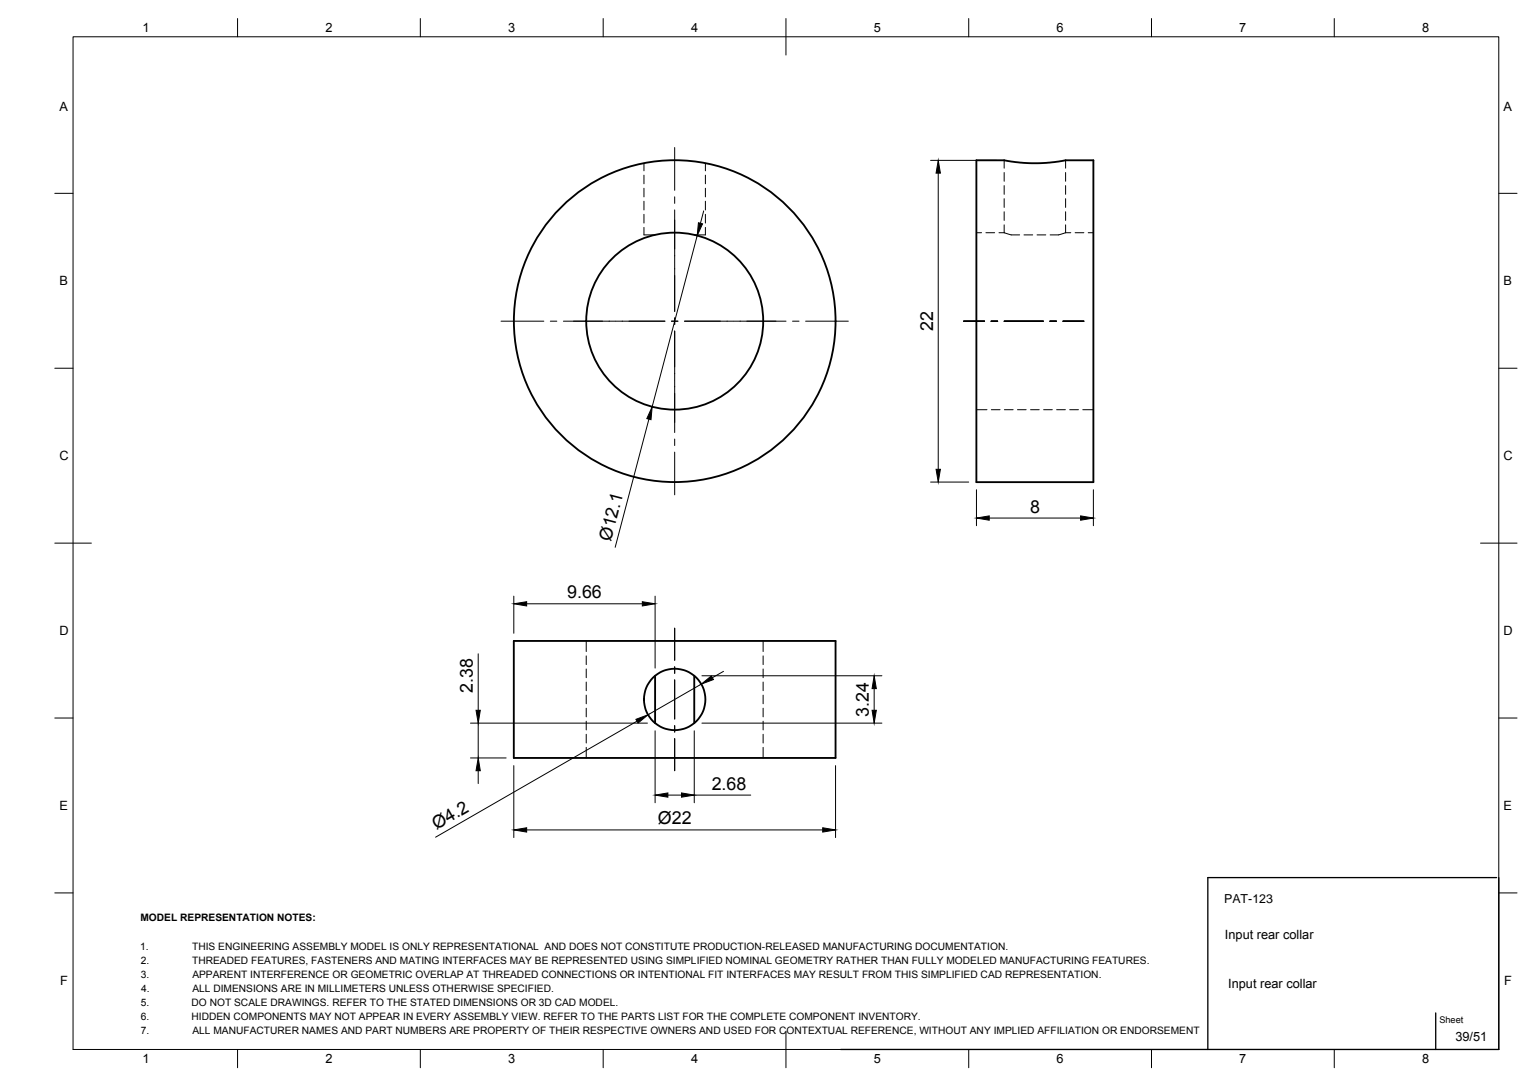
ISO-10303-21;
HEADER;
/* Generated by software containing ST-Developer
 * from STEP Tools, Inc. (www.steptools.com) 
 */

FILE_DESCRIPTION(
/* description */ ('Worm-less right-angle friction wheel drive'),
/* implementation_level */ '2;1');

FILE_NAME(
/* name */ 'Input rear collar.step',
/* time_stamp */ '2026-10-28T03:22:36-07:00',
/* author */ (''),
/* organization */ (''),
/* preprocessor_version */ 'ST-DEVELOPER v20.2',
/* originating_system */ 'Autodesk Translation Framework v15.17.0.0',
/* authorisation */ '');

FILE_SCHEMA (('AUTOMOTIVE_DESIGN { 1 0 10303 214 3 1 1 }'));
ENDSEC;

DATA;
#10=MECHANICAL_DESIGN_GEOMETRIC_PRESENTATION_REPRESENTATION('',(#652),#17046);
#497=B_SPLINE_CURVE_WITH_KNOTS('',3,(#16212,#16213,#16214,#16215,#16216,
#16217,#16218,#16219,#16220,#16221),.UNSPECIFIED.,.F.,.F.,(4,2,2,2,4),(0.818088904349172,
0.878131747417165,0.957937926194036,1.03774410497091,1.0977869480389),
 .UNSPECIFIED.);
#498=B_SPLINE_CURVE_WITH_KNOTS('',3,(#16227,#16228,#16229,#16230,#16231,
#16232,#16233,#16234,#16235,#16236,#16237,#16238,#16239,#16240,#16241,#16242,
#16243,#16244),.UNSPECIFIED.,.F.,.F.,(4,2,2,2,2,2,2,2,4),(0.,0.0793157643915219,
0.158631528783044,0.23794361593365,0.317255703084256,0.396567790234861,
0.475879877385467,0.555195641776989,0.634511406168511),.UNSPECIFIED.);
#499=B_SPLINE_CURVE_WITH_KNOTS('',3,(#16245,#16246,#16247,#16248,#16249,
#16250,#16251,#16252,#16253,#16254,#16255,#16256,#16257,#16258,#16259,#16260,
#16261,#16262),.UNSPECIFIED.,.F.,.F.,(4,2,2,2,2,2,2,2,4),(0.634511406168511,
0.713827170560033,0.793142934951555,0.872455022102161,0.951767109252766,
1.03107919640337,1.11039128355398,1.1897070479455,1.26902281233702),
 .UNSPECIFIED.);
#500=B_SPLINE_CURVE_WITH_KNOTS('',3,(#16265,#16266,#16267,#16268,#16269,
#16270,#16271,#16272,#16273,#16274),.UNSPECIFIED.,.F.,.F.,(4,2,2,2,4),(0.179463620219816,
0.239506463287808,0.319312642064679,0.399118820841549,0.459161663909541),
 .UNSPECIFIED.);
#551=SHAPE_REPRESENTATION_RELATIONSHIP('SRR','None',#17296,#598);
#598=ADVANCED_BREP_SHAPE_REPRESENTATION('',(#703),#17032);
#652=STYLED_ITEM('',(#17584),#703);
#703=MANIFOLD_SOLID_BREP('Body1',#8210);
#925=FACE_BOUND('',#2249,.T.);
#926=FACE_BOUND('',#2251,.T.);
#927=FACE_BOUND('',#2253,.T.);
#928=FACE_BOUND('',#2255,.T.);
#1137=PLANE('',#9491);
#1138=PLANE('',#9496);
#1139=PLANE('',#9503);
#1140=PLANE('',#9504);
#1569=FACE_OUTER_BOUND('',#2245,.T.);
#1570=FACE_OUTER_BOUND('',#2246,.T.);
#1571=FACE_OUTER_BOUND('',#2247,.T.);
#1572=FACE_OUTER_BOUND('',#2248,.T.);
#1573=FACE_OUTER_BOUND('',#2250,.T.);
#1574=FACE_OUTER_BOUND('',#2252,.T.);
#1575=FACE_OUTER_BOUND('',#2254,.T.);
#2245=EDGE_LOOP('',(#7098,#7099));
#2246=EDGE_LOOP('',(#7100,#7101,#7102,#7103,#7104,#7105,#7106,#7107,#7108));
#2247=EDGE_LOOP('',(#7109,#7110,#7111));
#2248=EDGE_LOOP('',(#7112,#7113,#7114,#7115));
#2249=EDGE_LOOP('',(#7116,#7117,#7118,#7119));
#2250=EDGE_LOOP('',(#7120,#7121,#7122,#7123));
#2251=EDGE_LOOP('',(#7124,#7125));
#2252=EDGE_LOOP('',(#7126));
#2253=EDGE_LOOP('',(#7127));
#2254=EDGE_LOOP('',(#7128));
#2255=EDGE_LOOP('',(#7129));
#2785=LINE('',#16208,#3325);
#2786=LINE('',#16225,#3326);
#2787=LINE('',#16276,#3327);
#2788=LINE('',#16281,#3328);
#2789=LINE('',#16287,#3329);
#3325=VECTOR('',#11681,1.);
#3326=VECTOR('',#11688,0.21);
#3327=VECTOR('',#11693,1.);
#3328=VECTOR('',#11698,0.605);
#3329=VECTOR('',#11705,1.1);
#3803=CIRCLE('',#9492,0.21);
#3804=CIRCLE('',#9494,0.21);
#3805=CIRCLE('',#9495,0.21);
#3806=CIRCLE('',#9498,0.605);
#3807=CIRCLE('',#9499,0.605);
#3808=CIRCLE('',#9501,1.1);
#3809=CIRCLE('',#9502,1.1);
#4394=VERTEX_POINT('',#16206);
#4395=VERTEX_POINT('',#16207);
#4396=VERTEX_POINT('',#16211);
#4397=VERTEX_POINT('',#16222);
#4398=VERTEX_POINT('',#16224);
#4399=VERTEX_POINT('',#16226);
#4400=VERTEX_POINT('',#16263);
#4401=VERTEX_POINT('',#16278);
#4402=VERTEX_POINT('',#16280);
#4403=VERTEX_POINT('',#16284);
#4404=VERTEX_POINT('',#16286);
#5318=EDGE_CURVE('',#4394,#4395,#2785,.T.);
#5319=EDGE_CURVE('',#4394,#4395,#3803,.T.);
#5320=EDGE_CURVE('',#4396,#4394,#497,.T.);
#5321=EDGE_CURVE('',#4397,#4396,#3804,.T.);
#5322=EDGE_CURVE('',#4397,#4398,#2786,.T.);
#5323=EDGE_CURVE('',#4399,#4398,#498,.T.);
#5324=EDGE_CURVE('',#4398,#4399,#499,.T.);
#5325=EDGE_CURVE('',#4400,#4397,#3805,.T.);
#5326=EDGE_CURVE('',#4395,#4400,#500,.T.);
#5327=EDGE_CURVE('',#4400,#4396,#2787,.T.);
#5328=EDGE_CURVE('',#4401,#4401,#3806,.T.);
#5329=EDGE_CURVE('',#4401,#4402,#2788,.T.);
#5330=EDGE_CURVE('',#4402,#4402,#3807,.T.);
#5331=EDGE_CURVE('',#4403,#4403,#3808,.T.);
#5332=EDGE_CURVE('',#4403,#4404,#2789,.T.);
#5333=EDGE_CURVE('',#4404,#4404,#3809,.T.);
#7098=ORIENTED_EDGE('',*,*,#5318,.F.);
#7099=ORIENTED_EDGE('',*,*,#5319,.T.);
#7100=ORIENTED_EDGE('',*,*,#5320,.F.);
#7101=ORIENTED_EDGE('',*,*,#5321,.F.);
#7102=ORIENTED_EDGE('',*,*,#5322,.T.);
#7103=ORIENTED_EDGE('',*,*,#5323,.F.);
#7104=ORIENTED_EDGE('',*,*,#5324,.F.);
#7105=ORIENTED_EDGE('',*,*,#5322,.F.);
#7106=ORIENTED_EDGE('',*,*,#5325,.F.);
#7107=ORIENTED_EDGE('',*,*,#5326,.F.);
#7108=ORIENTED_EDGE('',*,*,#5319,.F.);
#7109=ORIENTED_EDGE('',*,*,#5327,.F.);
#7110=ORIENTED_EDGE('',*,*,#5325,.T.);
#7111=ORIENTED_EDGE('',*,*,#5321,.T.);
#7112=ORIENTED_EDGE('',*,*,#5328,.F.);
#7113=ORIENTED_EDGE('',*,*,#5329,.T.);
#7114=ORIENTED_EDGE('',*,*,#5330,.T.);
#7115=ORIENTED_EDGE('',*,*,#5329,.F.);
#7116=ORIENTED_EDGE('',*,*,#5326,.T.);
#7117=ORIENTED_EDGE('',*,*,#5327,.T.);
#7118=ORIENTED_EDGE('',*,*,#5320,.T.);
#7119=ORIENTED_EDGE('',*,*,#5318,.T.);
#7120=ORIENTED_EDGE('',*,*,#5331,.F.);
#7121=ORIENTED_EDGE('',*,*,#5332,.T.);
#7122=ORIENTED_EDGE('',*,*,#5333,.T.);
#7123=ORIENTED_EDGE('',*,*,#5332,.F.);
#7124=ORIENTED_EDGE('',*,*,#5323,.T.);
#7125=ORIENTED_EDGE('',*,*,#5324,.T.);
#7126=ORIENTED_EDGE('',*,*,#5331,.T.);
#7127=ORIENTED_EDGE('',*,*,#5328,.T.);
#7128=ORIENTED_EDGE('',*,*,#5333,.F.);
#7129=ORIENTED_EDGE('',*,*,#5330,.F.);
#7671=CYLINDRICAL_SURFACE('',#9493,0.21);
#7672=CYLINDRICAL_SURFACE('',#9497,0.605);
#7673=CYLINDRICAL_SURFACE('',#9500,1.1);
#8061=ADVANCED_FACE('',(#1569),#1137,.T.);
#8062=ADVANCED_FACE('',(#1570),#7671,.F.);
#8063=ADVANCED_FACE('',(#1571),#1138,.T.);
#8064=ADVANCED_FACE('',(#1572,#925),#7672,.F.);
#8065=ADVANCED_FACE('',(#1573,#926),#7673,.T.);
#8066=ADVANCED_FACE('',(#1574,#927),#1139,.T.);
#8067=ADVANCED_FACE('',(#1575,#928),#1140,.F.);
#8210=CLOSED_SHELL('',(#8061,#8062,#8063,#8064,#8065,#8066,#8067));
#9490=AXIS2_PLACEMENT_3D('',#16204,#11677,#11678);
#9491=AXIS2_PLACEMENT_3D('',#16205,#11679,#11680);
#9492=AXIS2_PLACEMENT_3D('',#16209,#11682,#11683);
#9493=AXIS2_PLACEMENT_3D('',#16210,#11684,#11685);
#9494=AXIS2_PLACEMENT_3D('',#16223,#11686,#11687);
#9495=AXIS2_PLACEMENT_3D('',#16264,#11689,#11690);
#9496=AXIS2_PLACEMENT_3D('',#16275,#11691,#11692);
#9497=AXIS2_PLACEMENT_3D('',#16277,#11694,#11695);
#9498=AXIS2_PLACEMENT_3D('',#16279,#11696,#11697);
#9499=AXIS2_PLACEMENT_3D('',#16282,#11699,#11700);
#9500=AXIS2_PLACEMENT_3D('',#16283,#11701,#11702);
#9501=AXIS2_PLACEMENT_3D('',#16285,#11703,#11704);
#9502=AXIS2_PLACEMENT_3D('',#16288,#11706,#11707);
#9503=AXIS2_PLACEMENT_3D('',#16289,#11708,#11709);
#9504=AXIS2_PLACEMENT_3D('',#16290,#11710,#11711);
#11677=DIRECTION('axis',(0.,0.,1.));
#11678=DIRECTION('refdir',(1.,0.,0.));
#11679=DIRECTION('center_axis',(0.,0.,1.));
#11680=DIRECTION('ref_axis',(1.,0.,0.));
#11681=DIRECTION('',(0.,1.,0.));
#11682=DIRECTION('center_axis',(0.,0.,1.));
#11683=DIRECTION('ref_axis',(1.,0.,0.));
#11684=DIRECTION('center_axis',(0.,0.,1.));
#11685=DIRECTION('ref_axis',(1.,0.,0.));
#11686=DIRECTION('center_axis',(0.,0.,1.));
#11687=DIRECTION('ref_axis',(1.,0.,0.));
#11688=DIRECTION('',(0.,0.,1.));
#11689=DIRECTION('center_axis',(0.,0.,1.));
#11690=DIRECTION('ref_axis',(1.,0.,0.));
#11691=DIRECTION('center_axis',(0.,0.,1.));
#11692=DIRECTION('ref_axis',(1.,0.,0.));
#11693=DIRECTION('',(0.,-1.,0.));
#11694=DIRECTION('center_axis',(0.,1.,0.));
#11695=DIRECTION('ref_axis',(1.,0.,0.));
#11696=DIRECTION('center_axis',(0.,-1.,0.));
#11697=DIRECTION('ref_axis',(1.,0.,0.));
#11698=DIRECTION('',(0.,-1.,0.));
#11699=DIRECTION('center_axis',(0.,-1.,0.));
#11700=DIRECTION('ref_axis',(1.,0.,0.));
#11701=DIRECTION('center_axis',(0.,1.,0.));
#11702=DIRECTION('ref_axis',(1.,0.,0.));
#11703=DIRECTION('center_axis',(0.,1.,0.));
#11704=DIRECTION('ref_axis',(1.,0.,0.));
#11705=DIRECTION('',(0.,-1.,0.));
#11706=DIRECTION('center_axis',(0.,1.,0.));
#11707=DIRECTION('ref_axis',(1.,0.,0.));
#11708=DIRECTION('center_axis',(0.,1.,0.));
#11709=DIRECTION('ref_axis',(1.,0.,0.));
#11710=DIRECTION('center_axis',(0.,1.,0.));
#11711=DIRECTION('ref_axis',(1.,0.,0.));
#16204=CARTESIAN_POINT('',(0.,0.,0.));
#16205=CARTESIAN_POINT('Origin',(0.,-7.9,7.59));
#16206=CARTESIAN_POINT('',(0.133884278389956,-8.06178689687364,7.59));
#16207=CARTESIAN_POINT('',(0.133884278389956,-7.73821310312636,7.59));
#16208=CARTESIAN_POINT('',(0.133884278389956,-8.3,7.59));
#16209=CARTESIAN_POINT('Origin',(0.,-7.9,7.59));
#16210=CARTESIAN_POINT('Origin',(0.,-7.9,7.59));
#16211=CARTESIAN_POINT('',(-0.133884278389956,-8.06178689687364,7.59));
#16212=CARTESIAN_POINT('Ctrl Pts',(-0.133884278389956,-8.06178689687364,
7.59));
#16213=CARTESIAN_POINT('Ctrl Pts',(-0.118254395260802,-8.07472116821763,
7.59354677224418));
#16214=CARTESIAN_POINT('Ctrl Pts',(-0.100109787682299,-8.08579931658744,
7.59698224789957));
#16215=CARTESIAN_POINT('Ctrl Pts',(-0.054829872132519,-8.10463856105443,
7.6030741628997));
#16216=CARTESIAN_POINT('Ctrl Pts',(-0.0266020595922904,-8.11,7.605));
#16217=CARTESIAN_POINT('Ctrl Pts',(0.0266020595922903,-8.11,7.605));
#16218=CARTESIAN_POINT('Ctrl Pts',(0.0548298721325189,-8.10463856105443,
7.6030741628997));
#16219=CARTESIAN_POINT('Ctrl Pts',(0.100109787682299,-8.08579931658744,
7.59698224789957));
#16220=CARTESIAN_POINT('Ctrl Pts',(0.118254395260802,-8.07472116821763,
7.59354677224418));
#16221=CARTESIAN_POINT('Ctrl Pts',(0.133884278389957,-8.06178689687364,
7.59));
#16222=CARTESIAN_POINT('',(-0.21,-7.9,7.59));
#16223=CARTESIAN_POINT('Origin',(0.,-7.9,7.59));
#16224=CARTESIAN_POINT('',(-0.21,-7.9,8.07976849370594));
#16225=CARTESIAN_POINT('',(-0.21,-7.9,7.59));
#16226=CARTESIAN_POINT('',(0.21,-7.9,8.07976849370594));
#16227=CARTESIAN_POINT('Ctrl Pts',(0.21,-7.9,8.07976849370594));
#16228=CARTESIAN_POINT('Ctrl Pts',(0.21,-7.92643858813051,8.07976849370594));
#16229=CARTESIAN_POINT('Ctrl Pts',(0.204702922670977,-7.95459378125493,
8.08084015664674));
#16230=CARTESIAN_POINT('Ctrl Pts',(0.183251796806355,-8.00631344554134,
8.08468313707126));
#16231=CARTESIAN_POINT('Ctrl Pts',(0.167101177357214,-8.02988367074114,
8.08739593054622));
#16232=CARTESIAN_POINT('Ctrl Pts',(0.129884533480965,-8.06710031461738,
8.09246633289124));
#16233=CARTESIAN_POINT('Ctrl Pts',(0.106313940757289,-8.08325161016341,
8.09515738895358));
#16234=CARTESIAN_POINT('Ctrl Pts',(0.0545930033295209,-8.10470322656974,
8.09895039220591));
#16235=CARTESIAN_POINT('Ctrl Pts',(0.0264373623835353,-8.11,8.1));
#16236=CARTESIAN_POINT('Ctrl Pts',(-0.0264373623835353,-8.11,8.1));
#16237=CARTESIAN_POINT('Ctrl Pts',(-0.0545930033295208,-8.10470322656974,
8.09895039220591));
#16238=CARTESIAN_POINT('Ctrl Pts',(-0.106313940757289,-8.08325161016341,
8.09515738895358));
#16239=CARTESIAN_POINT('Ctrl Pts',(-0.129884533480965,-8.06710031461738,
8.09246633289124));
#16240=CARTESIAN_POINT('Ctrl Pts',(-0.167101177357214,-8.02988367074114,
8.08739593054622));
#16241=CARTESIAN_POINT('Ctrl Pts',(-0.183251796806355,-8.00631344554134,
8.08468313707126));
#16242=CARTESIAN_POINT('Ctrl Pts',(-0.204702922670977,-7.95459378125493,
8.08084015664674));
#16243=CARTESIAN_POINT('Ctrl Pts',(-0.21,-7.92643858813051,8.07976849370594));
#16244=CARTESIAN_POINT('Ctrl Pts',(-0.21,-7.9,8.07976849370594));
#16245=CARTESIAN_POINT('Ctrl Pts',(-0.21,-7.9,8.07976849370594));
#16246=CARTESIAN_POINT('Ctrl Pts',(-0.21,-7.87356141186949,8.07976849370594));
#16247=CARTESIAN_POINT('Ctrl Pts',(-0.204702922670977,-7.84540621874507,
8.08084015664674));
#16248=CARTESIAN_POINT('Ctrl Pts',(-0.183251796806355,-7.79368655445866,
8.08468313707126));
#16249=CARTESIAN_POINT('Ctrl Pts',(-0.167101177357215,-7.77011632925886,
8.08739593054622));
#16250=CARTESIAN_POINT('Ctrl Pts',(-0.129884533480965,-7.73289968538262,
8.09246633289124));
#16251=CARTESIAN_POINT('Ctrl Pts',(-0.106313940757289,-7.71674838983659,
8.09515738895358));
#16252=CARTESIAN_POINT('Ctrl Pts',(-0.054593003329521,-7.69529677343026,
8.09895039220591));
#16253=CARTESIAN_POINT('Ctrl Pts',(-0.0264373623835353,-7.69,8.1));
#16254=CARTESIAN_POINT('Ctrl Pts',(0.0264373623835353,-7.69,8.1));
#16255=CARTESIAN_POINT('Ctrl Pts',(0.0545930033295201,-7.69529677343026,
8.09895039220591));
#16256=CARTESIAN_POINT('Ctrl Pts',(0.106313940757288,-7.71674838983659,
8.09515738895358));
#16257=CARTESIAN_POINT('Ctrl Pts',(0.129884533480965,-7.73289968538262,
8.09246633289124));
#16258=CARTESIAN_POINT('Ctrl Pts',(0.167101177357214,-7.77011632925886,
8.08739593054622));
#16259=CARTESIAN_POINT('Ctrl Pts',(0.183251796806355,-7.79368655445866,
8.08468313707126));
#16260=CARTESIAN_POINT('Ctrl Pts',(0.204702922670977,-7.84540621874507,
8.08084015664674));
#16261=CARTESIAN_POINT('Ctrl Pts',(0.21,-7.87356141186949,8.07976849370594));
#16262=CARTESIAN_POINT('Ctrl Pts',(0.21,-7.9,8.07976849370594));
#16263=CARTESIAN_POINT('',(-0.133884278389956,-7.73821310312636,7.59));
#16264=CARTESIAN_POINT('Origin',(0.,-7.9,7.59));
#16265=CARTESIAN_POINT('Ctrl Pts',(0.133884278389956,-7.73821310312636,
7.59));
#16266=CARTESIAN_POINT('Ctrl Pts',(0.118254395260802,-7.72527883178237,
7.59354677224418));
#16267=CARTESIAN_POINT('Ctrl Pts',(0.100109787682299,-7.71420068341256,
7.59698224789957));
#16268=CARTESIAN_POINT('Ctrl Pts',(0.0548298721325194,-7.69536143894557,
7.6030741628997));
#16269=CARTESIAN_POINT('Ctrl Pts',(0.0266020595922903,-7.69,7.605));
#16270=CARTESIAN_POINT('Ctrl Pts',(-0.0266020595922902,-7.69,7.605));
#16271=CARTESIAN_POINT('Ctrl Pts',(-0.0548298721325196,-7.69536143894557,
7.6030741628997));
#16272=CARTESIAN_POINT('Ctrl Pts',(-0.100109787682299,-7.71420068341256,
7.59698224789957));
#16273=CARTESIAN_POINT('Ctrl Pts',(-0.118254395260801,-7.72527883178237,
7.59354677224418));
#16274=CARTESIAN_POINT('Ctrl Pts',(-0.133884278389955,-7.73821310312636,
7.59));
#16275=CARTESIAN_POINT('Origin',(0.,-7.9,7.59));
#16276=CARTESIAN_POINT('',(-0.133884278389956,-8.3,7.59));
#16277=CARTESIAN_POINT('Origin',(0.,-8.3,7.));
#16278=CARTESIAN_POINT('',(-0.605,-7.5,7.));
#16279=CARTESIAN_POINT('Origin',(0.,-7.5,7.));
#16280=CARTESIAN_POINT('',(-0.605,-8.3,7.));
#16281=CARTESIAN_POINT('',(-0.605,-8.3,7.));
#16282=CARTESIAN_POINT('Origin',(0.,-8.3,7.));
#16283=CARTESIAN_POINT('Origin',(0.,-8.3,7.));
#16284=CARTESIAN_POINT('',(-1.1,-7.5,7.));
#16285=CARTESIAN_POINT('Origin',(0.,-7.5,7.));
#16286=CARTESIAN_POINT('',(-1.1,-8.3,7.));
#16287=CARTESIAN_POINT('',(-1.1,-8.3,7.));
#16288=CARTESIAN_POINT('Origin',(0.,-8.3,7.));
#16289=CARTESIAN_POINT('Origin',(0.,-7.5,7.));
#16290=CARTESIAN_POINT('Origin',(0.,-8.3,7.));
#16979=UNCERTAINTY_MEASURE_WITH_UNIT(LENGTH_MEASURE(0.001),#17047,
'DISTANCE_ACCURACY_VALUE',
'Maximum model space distance between geometric entities at asserted c
onnectivities');
#16993=UNCERTAINTY_MEASURE_WITH_UNIT(LENGTH_MEASURE(0.001),#17047,
'DISTANCE_ACCURACY_VALUE',
'Maximum model space distance between geometric entities at asserted c
onnectivities');
#17032=(
GEOMETRIC_REPRESENTATION_CONTEXT(3)
GLOBAL_UNCERTAINTY_ASSIGNED_CONTEXT((#16979))
GLOBAL_UNIT_ASSIGNED_CONTEXT((#17047,#17049,#17050))
REPRESENTATION_CONTEXT('','3D')
);
#17046=(
GEOMETRIC_REPRESENTATION_CONTEXT(3)
GLOBAL_UNCERTAINTY_ASSIGNED_CONTEXT((#16993))
GLOBAL_UNIT_ASSIGNED_CONTEXT((#17047,#17049,#17050))
REPRESENTATION_CONTEXT('','3D')
);
#17047=(
LENGTH_UNIT()
NAMED_UNIT(*)
SI_UNIT(.CENTI.,.METRE.)
);
#17049=(
NAMED_UNIT(*)
PLANE_ANGLE_UNIT()
SI_UNIT($,.RADIAN.)
);
#17050=(
NAMED_UNIT(*)
SI_UNIT($,.STERADIAN.)
SOLID_ANGLE_UNIT()
);
#17089=SHAPE_DEFINITION_REPRESENTATION(#17146,#17296);
#17146=PRODUCT_DEFINITION_SHAPE('',$,#17349);
#17296=SHAPE_REPRESENTATION('',(#9490),#17032);
#17310=PRODUCT_DEFINITION_CONTEXT('part definition',#17468,'design');
#17349=PRODUCT_DEFINITION('Input rear collar','Input rear collar',#17401,
#17310);
#17401=PRODUCT_DEFINITION_FORMATION('',$,#17508);
#17468=APPLICATION_CONTEXT(
'Core Data for Automotive Mechanical Design Process');
#17469=PRODUCT_CONTEXT('part definition',#17468,'mechanical');
#17508=PRODUCT('Input rear collar','Input rear collar',
'Input rear collar',(#17469));
#17578=COLOUR_RGB('Sky Blue',0.24,0.69,0.87);
#17579=FILL_AREA_STYLE_COLOUR('',#17578);
#17580=FILL_AREA_STYLE('',(#17579));
#17581=SURFACE_STYLE_FILL_AREA(#17580);
#17582=SURFACE_SIDE_STYLE('',(#17581));
#17583=SURFACE_STYLE_USAGE(.BOTH.,#17582);
#17584=PRESENTATION_STYLE_ASSIGNMENT((#17583));
ENDSEC;
END-ISO-10303-21;
